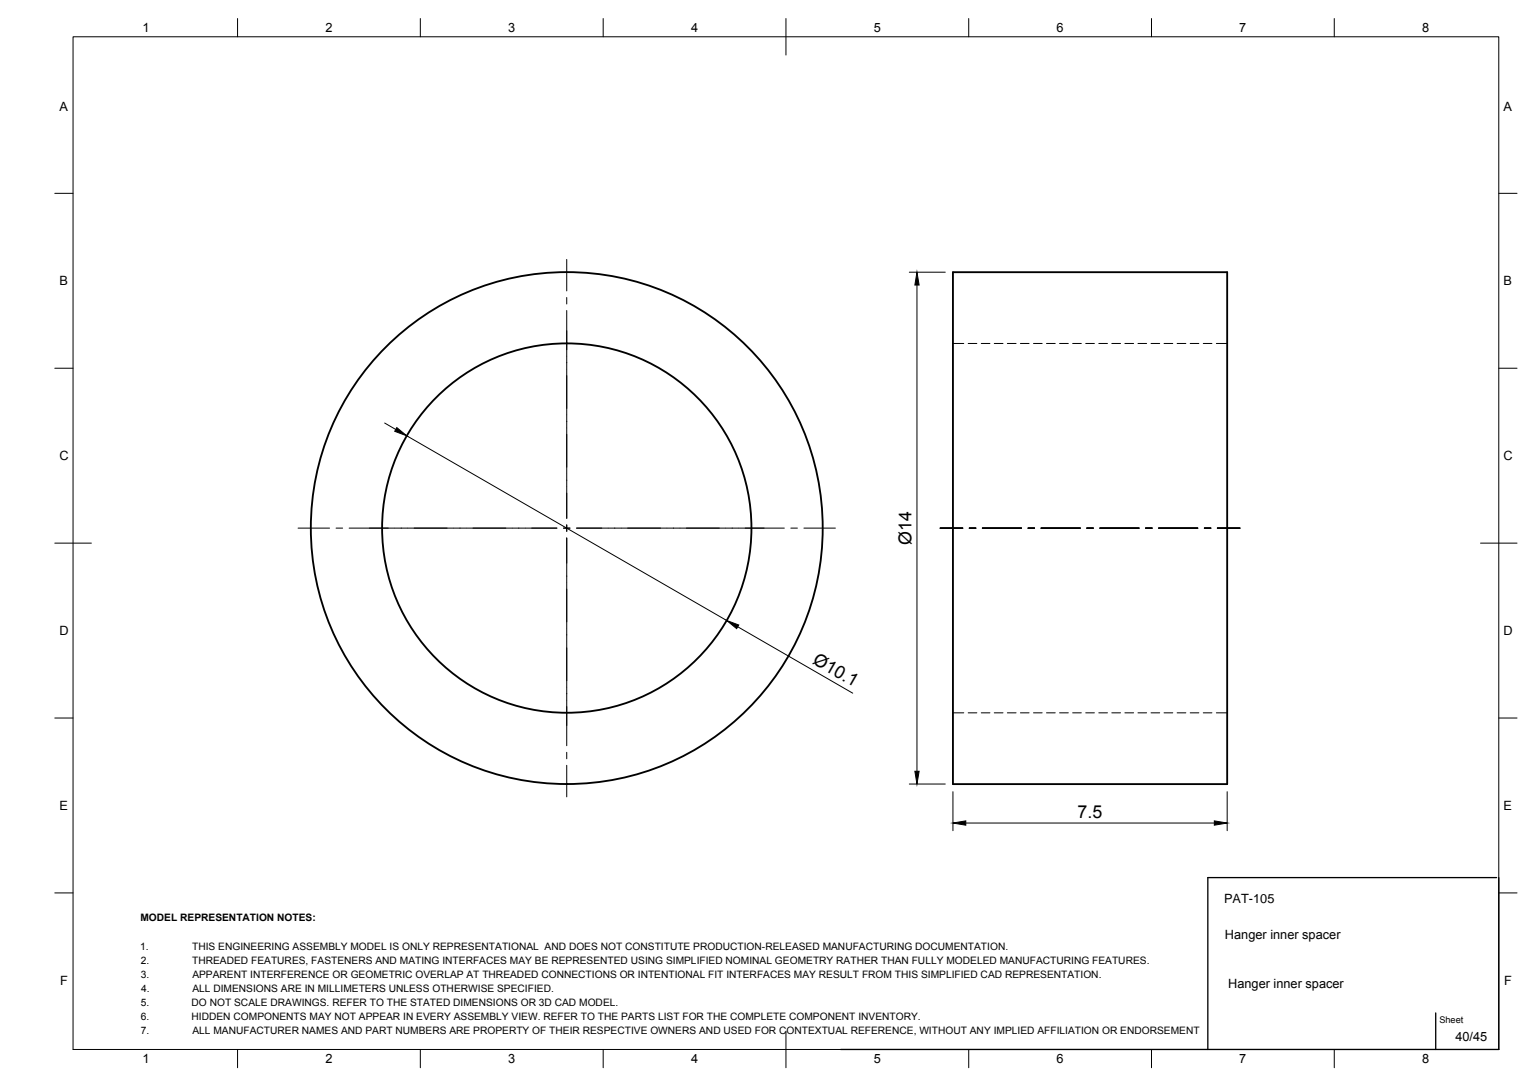
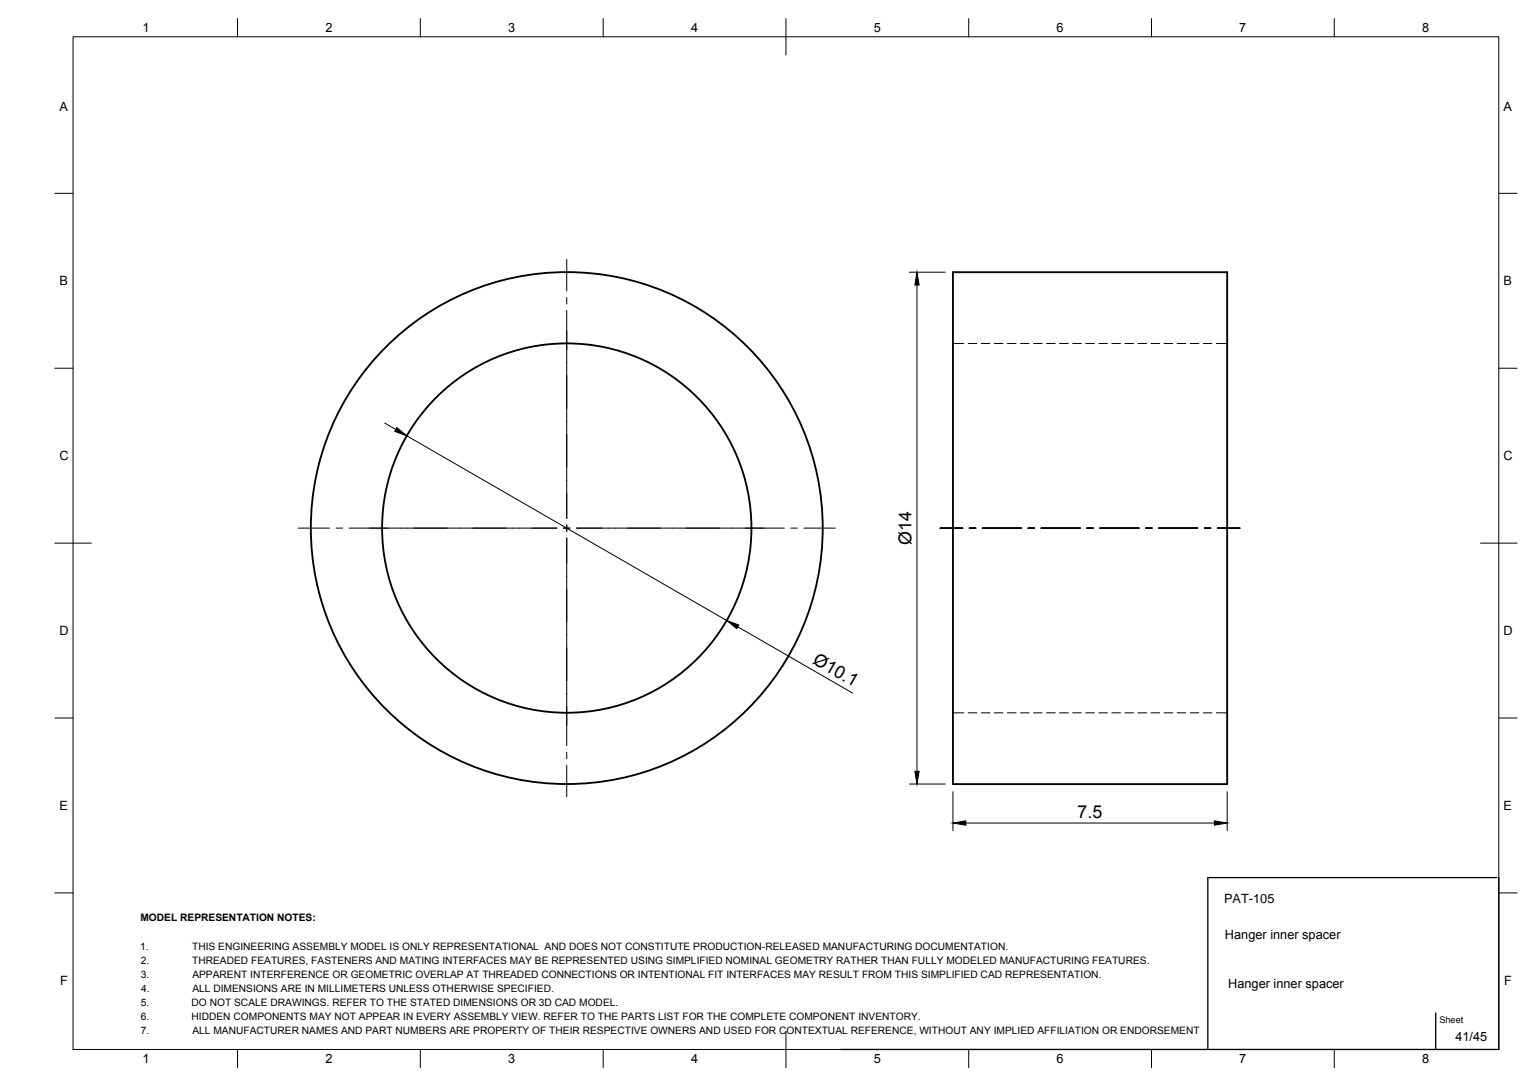
ISO-10303-21;
HEADER;
/* Generated by software containing ST-Developer
 * from STEP Tools, Inc. (www.steptools.com) 
 */

FILE_DESCRIPTION(
/* description */ ('Torque wrench calibration arm'),
/* implementation_level */ '2;1');

FILE_NAME(
/* name */ 'Hanger inner spacer.step',
/* time_stamp */ '2026-10-28T03:24:52-07:00',
/* author */ (''),
/* organization */ (''),
/* preprocessor_version */ 'ST-DEVELOPER v20.2',
/* originating_system */ 'Autodesk Translation Framework v15.17.0.0',
/* authorisation */ '');

FILE_SCHEMA (('AUTOMOTIVE_DESIGN { 1 0 10303 214 3 1 1 }'));
ENDSEC;

DATA;
#10=MECHANICAL_DESIGN_GEOMETRIC_PRESENTATION_REPRESENTATION('',(#473),#12783);
#382=SHAPE_REPRESENTATION_RELATIONSHIP('SRR','None',#12967,#419);
#419=ADVANCED_BREP_SHAPE_REPRESENTATION('',(#525),#12776);
#473=STYLED_ITEM('',(#13205),#525);
#525=MANIFOLD_SOLID_BREP('Body1',#6544);
#639=FACE_BOUND('',#1736,.T.);
#640=FACE_BOUND('',#1738,.T.);
#852=PLANE('',#7726);
#853=PLANE('',#7727);
#1230=FACE_OUTER_BOUND('',#1733,.T.);
#1231=FACE_OUTER_BOUND('',#1734,.T.);
#1232=FACE_OUTER_BOUND('',#1735,.T.);
#1233=FACE_OUTER_BOUND('',#1737,.T.);
#1733=EDGE_LOOP('',(#5855,#5856,#5857,#5858));
#1734=EDGE_LOOP('',(#5859,#5860,#5861,#5862));
#1735=EDGE_LOOP('',(#5863));
#1736=EDGE_LOOP('',(#5864));
#1737=EDGE_LOOP('',(#5865));
#1738=EDGE_LOOP('',(#5866));
#2166=LINE('',#12532,#2581);
#2167=LINE('',#12538,#2582);
#2581=VECTOR('',#9714,0.505000000000003);
#2582=VECTOR('',#9721,0.700000000000003);
#2940=CIRCLE('',#7721,0.505000000000003);
#2941=CIRCLE('',#7722,0.505000000000003);
#2942=CIRCLE('',#7724,0.700000000000003);
#2943=CIRCLE('',#7725,0.700000000000003);
#3490=VERTEX_POINT('',#12529);
#3491=VERTEX_POINT('',#12531);
#3492=VERTEX_POINT('',#12535);
#3493=VERTEX_POINT('',#12537);
#4285=EDGE_CURVE('',#3490,#3490,#2940,.T.);
#4286=EDGE_CURVE('',#3490,#3491,#2166,.T.);
#4287=EDGE_CURVE('',#3491,#3491,#2941,.T.);
#4288=EDGE_CURVE('',#3492,#3492,#2942,.T.);
#4289=EDGE_CURVE('',#3492,#3493,#2167,.T.);
#4290=EDGE_CURVE('',#3493,#3493,#2943,.T.);
#5855=ORIENTED_EDGE('',*,*,#4285,.F.);
#5856=ORIENTED_EDGE('',*,*,#4286,.T.);
#5857=ORIENTED_EDGE('',*,*,#4287,.T.);
#5858=ORIENTED_EDGE('',*,*,#4286,.F.);
#5859=ORIENTED_EDGE('',*,*,#4288,.F.);
#5860=ORIENTED_EDGE('',*,*,#4289,.T.);
#5861=ORIENTED_EDGE('',*,*,#4290,.T.);
#5862=ORIENTED_EDGE('',*,*,#4289,.F.);
#5863=ORIENTED_EDGE('',*,*,#4288,.T.);
#5864=ORIENTED_EDGE('',*,*,#4285,.T.);
#5865=ORIENTED_EDGE('',*,*,#4290,.F.);
#5866=ORIENTED_EDGE('',*,*,#4287,.F.);
#6086=CYLINDRICAL_SURFACE('',#7720,0.505000000000003);
#6087=CYLINDRICAL_SURFACE('',#7723,0.700000000000003);
#6455=ADVANCED_FACE('',(#1230),#6086,.F.);
#6456=ADVANCED_FACE('',(#1231),#6087,.T.);
#6457=ADVANCED_FACE('',(#1232,#639),#852,.T.);
#6458=ADVANCED_FACE('',(#1233,#640),#853,.F.);
#6544=CLOSED_SHELL('',(#6455,#6456,#6457,#6458));
#7719=AXIS2_PLACEMENT_3D('',#12527,#9708,#9709);
#7720=AXIS2_PLACEMENT_3D('',#12528,#9710,#9711);
#7721=AXIS2_PLACEMENT_3D('',#12530,#9712,#9713);
#7722=AXIS2_PLACEMENT_3D('',#12533,#9715,#9716);
#7723=AXIS2_PLACEMENT_3D('',#12534,#9717,#9718);
#7724=AXIS2_PLACEMENT_3D('',#12536,#9719,#9720);
#7725=AXIS2_PLACEMENT_3D('',#12539,#9722,#9723);
#7726=AXIS2_PLACEMENT_3D('',#12540,#9724,#9725);
#7727=AXIS2_PLACEMENT_3D('',#12541,#9726,#9727);
#9708=DIRECTION('axis',(0.,0.,1.));
#9709=DIRECTION('refdir',(1.,0.,0.));
#9710=DIRECTION('center_axis',(0.,1.,0.));
#9711=DIRECTION('ref_axis',(1.,0.,0.));
#9712=DIRECTION('center_axis',(0.,-1.,0.));
#9713=DIRECTION('ref_axis',(1.,0.,0.));
#9714=DIRECTION('',(0.,-1.,0.));
#9715=DIRECTION('center_axis',(0.,-1.,0.));
#9716=DIRECTION('ref_axis',(1.,0.,0.));
#9717=DIRECTION('center_axis',(0.,1.,0.));
#9718=DIRECTION('ref_axis',(1.,0.,0.));
#9719=DIRECTION('center_axis',(0.,1.,0.));
#9720=DIRECTION('ref_axis',(1.,0.,0.));
#9721=DIRECTION('',(0.,-1.,0.));
#9722=DIRECTION('center_axis',(0.,1.,0.));
#9723=DIRECTION('ref_axis',(1.,0.,0.));
#9724=DIRECTION('center_axis',(0.,1.,0.));
#9725=DIRECTION('ref_axis',(1.,0.,0.));
#9726=DIRECTION('center_axis',(0.,1.,0.));
#9727=DIRECTION('ref_axis',(1.,0.,0.));
#12527=CARTESIAN_POINT('',(0.,0.,0.));
#12528=CARTESIAN_POINT('Origin',(50.,7.3,8.));
#12529=CARTESIAN_POINT('',(49.495,8.05,8.));
#12530=CARTESIAN_POINT('Origin',(50.,8.05,8.));
#12531=CARTESIAN_POINT('',(49.495,7.3,8.));
#12532=CARTESIAN_POINT('',(49.495,7.3,8.));
#12533=CARTESIAN_POINT('Origin',(50.,7.3,8.));
#12534=CARTESIAN_POINT('Origin',(50.,7.3,8.));
#12535=CARTESIAN_POINT('',(49.3,8.05,8.));
#12536=CARTESIAN_POINT('Origin',(50.,8.05,8.));
#12537=CARTESIAN_POINT('',(49.3,7.3,8.));
#12538=CARTESIAN_POINT('',(49.3,7.3,8.));
#12539=CARTESIAN_POINT('Origin',(50.,7.3,8.));
#12540=CARTESIAN_POINT('Origin',(50.,8.05,8.));
#12541=CARTESIAN_POINT('Origin',(50.,7.3,8.));
#12732=UNCERTAINTY_MEASURE_WITH_UNIT(LENGTH_MEASURE(0.001),#12784,
'DISTANCE_ACCURACY_VALUE',
'Maximum model space distance between geometric entities at asserted c
onnectivities');
#12739=UNCERTAINTY_MEASURE_WITH_UNIT(LENGTH_MEASURE(0.001),#12784,
'DISTANCE_ACCURACY_VALUE',
'Maximum model space distance between geometric entities at asserted c
onnectivities');
#12776=(
GEOMETRIC_REPRESENTATION_CONTEXT(3)
GLOBAL_UNCERTAINTY_ASSIGNED_CONTEXT((#12732))
GLOBAL_UNIT_ASSIGNED_CONTEXT((#12784,#12786,#12787))
REPRESENTATION_CONTEXT('','3D')
);
#12783=(
GEOMETRIC_REPRESENTATION_CONTEXT(3)
GLOBAL_UNCERTAINTY_ASSIGNED_CONTEXT((#12739))
GLOBAL_UNIT_ASSIGNED_CONTEXT((#12784,#12786,#12787))
REPRESENTATION_CONTEXT('','3D')
);
#12784=(
LENGTH_UNIT()
NAMED_UNIT(*)
SI_UNIT(.CENTI.,.METRE.)
);
#12786=(
NAMED_UNIT(*)
PLANE_ANGLE_UNIT()
SI_UNIT($,.RADIAN.)
);
#12787=(
NAMED_UNIT(*)
SI_UNIT($,.STERADIAN.)
SOLID_ANGLE_UNIT()
);
#12824=SHAPE_DEFINITION_REPRESENTATION(#12911,#12967);
#12911=PRODUCT_DEFINITION_SHAPE('',$,#13011);
#12967=SHAPE_REPRESENTATION('',(#7719),#12776);
#12974=PRODUCT_DEFINITION_CONTEXT('part definition',#13105,'design');
#13011=PRODUCT_DEFINITION('Hanger inner spacer','Hanger inner spacer',#13054,
#12974);
#13054=PRODUCT_DEFINITION_FORMATION('',$,#13143);
#13105=APPLICATION_CONTEXT(
'Core Data for Automotive Mechanical Design Process');
#13106=PRODUCT_CONTEXT('part definition',#13105,'mechanical');
#13143=PRODUCT('Hanger inner spacer','Hanger inner spacer',
'Hanger inner spacer',(#13106));
#13199=COLOUR_RGB('Sky Blue',0.24,0.69,0.87);
#13200=FILL_AREA_STYLE_COLOUR('',#13199);
#13201=FILL_AREA_STYLE('',(#13200));
#13202=SURFACE_STYLE_FILL_AREA(#13201);
#13203=SURFACE_SIDE_STYLE('',(#13202));
#13204=SURFACE_STYLE_USAGE(.BOTH.,#13203);
#13205=PRESENTATION_STYLE_ASSIGNMENT((#13204));
ENDSEC;
END-ISO-10303-21;
